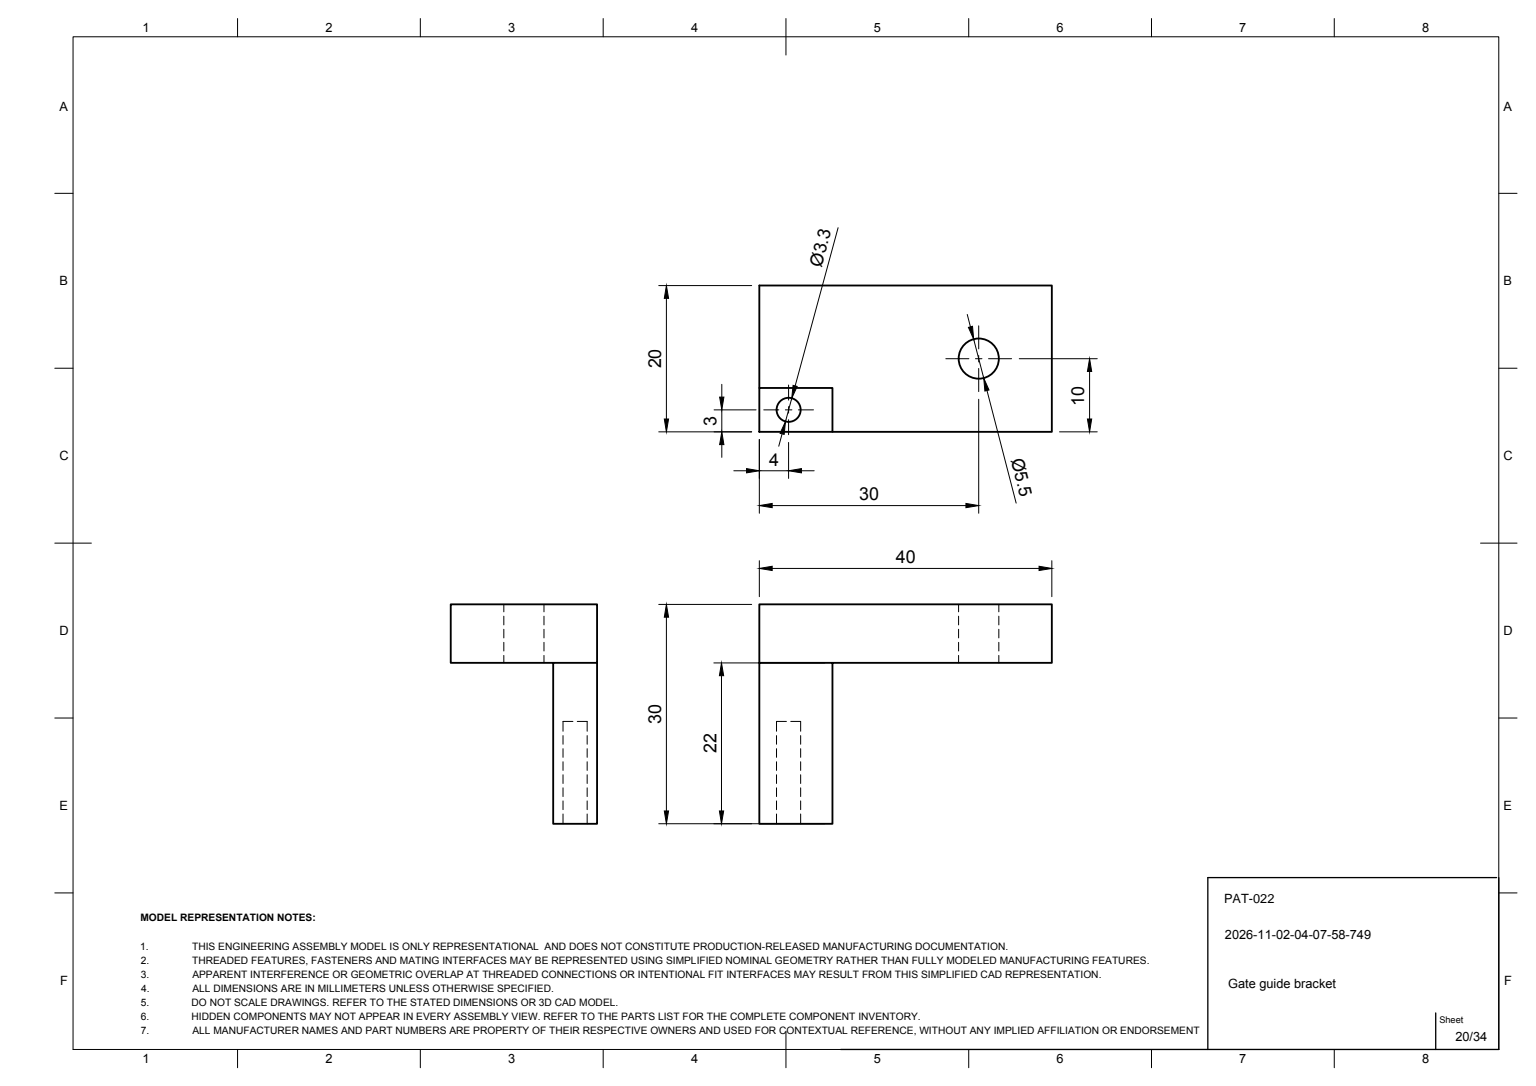
ISO-10303-21;
HEADER;
/* Generated by software containing ST-Developer
 * from STEP Tools, Inc. (www.steptools.com) 
 */

FILE_DESCRIPTION(
/* description */ ('Chute with adjustable gate'),
/* implementation_level */ '2;1');

FILE_NAME(
/* name */ 'Gate guide bracket.step',
/* time_stamp */ '2026-10-27T10:52:28-07:00',
/* author */ (''),
/* organization */ (''),
/* preprocessor_version */ 'ST-DEVELOPER v20.2',
/* originating_system */ 'Autodesk Translation Framework v15.17.0.0',
/* authorisation */ '');

FILE_SCHEMA (('AUTOMOTIVE_DESIGN { 1 0 10303 214 3 1 1 }'));
ENDSEC;

DATA;
#10=MECHANICAL_DESIGN_GEOMETRIC_PRESENTATION_REPRESENTATION('',(#429),#13094);
#365=SHAPE_REPRESENTATION_RELATIONSHIP('SRR','None',#13266,#397);
#397=ADVANCED_BREP_SHAPE_REPRESENTATION('',(#461),#13075);
#429=STYLED_ITEM('',(#13474),#461);
#461=MANIFOLD_SOLID_BREP('Body1',#7612);
#540=FACE_BOUND('',#1546,.T.);
#541=FACE_BOUND('',#1551,.T.);
#542=FACE_BOUND('',#1554,.T.);
#702=PLANE('',#8221);
#703=PLANE('',#8225);
#704=PLANE('',#8226);
#705=PLANE('',#8227);
#706=PLANE('',#8228);
#707=PLANE('',#8229);
#708=PLANE('',#8230);
#709=PLANE('',#8231);
#710=PLANE('',#8232);
#711=PLANE('',#8233);
#1060=FACE_OUTER_BOUND('',#1541,.T.);
#1061=FACE_OUTER_BOUND('',#1542,.T.);
#1062=FACE_OUTER_BOUND('',#1543,.T.);
#1063=FACE_OUTER_BOUND('',#1544,.T.);
#1064=FACE_OUTER_BOUND('',#1545,.T.);
#1065=FACE_OUTER_BOUND('',#1547,.T.);
#1066=FACE_OUTER_BOUND('',#1548,.T.);
#1067=FACE_OUTER_BOUND('',#1549,.T.);
#1068=FACE_OUTER_BOUND('',#1550,.T.);
#1069=FACE_OUTER_BOUND('',#1552,.T.);
#1070=FACE_OUTER_BOUND('',#1553,.T.);
#1071=FACE_OUTER_BOUND('',#1555,.T.);
#1541=EDGE_LOOP('',(#5834,#5835,#5836,#5837));
#1542=EDGE_LOOP('',(#5838));
#1543=EDGE_LOOP('',(#5839,#5840,#5841,#5842));
#1544=EDGE_LOOP('',(#5843,#5844,#5845,#5846));
#1545=EDGE_LOOP('',(#5847,#5848,#5849,#5850));
#1546=EDGE_LOOP('',(#5851));
#1547=EDGE_LOOP('',(#5852,#5853,#5854,#5855));
#1548=EDGE_LOOP('',(#5856,#5857,#5858,#5859,#5860,#5861));
#1549=EDGE_LOOP('',(#5862,#5863,#5864,#5865,#5866,#5867));
#1550=EDGE_LOOP('',(#5868,#5869,#5870,#5871));
#1551=EDGE_LOOP('',(#5872));
#1552=EDGE_LOOP('',(#5873,#5874,#5875,#5876));
#1553=EDGE_LOOP('',(#5877,#5878,#5879,#5880,#5881,#5882));
#1554=EDGE_LOOP('',(#5883));
#1555=EDGE_LOOP('',(#5884,#5885,#5886,#5887));
#2116=LINE('',#11607,#2893);
#2117=LINE('',#11614,#2894);
#2118=LINE('',#11619,#2895);
#2119=LINE('',#11621,#2896);
#2120=LINE('',#11623,#2897);
#2121=LINE('',#11624,#2898);
#2122=LINE('',#11627,#2899);
#2123=LINE('',#11629,#2900);
#2124=LINE('',#11630,#2901);
#2125=LINE('',#11633,#2902);
#2126=LINE('',#11634,#2903);
#2127=LINE('',#11637,#2904);
#2128=LINE('',#11639,#2905);
#2129=LINE('',#11641,#2906);
#2130=LINE('',#11642,#2907);
#2131=LINE('',#11645,#2908);
#2132=LINE('',#11647,#2909);
#2133=LINE('',#11648,#2910);
#2134=LINE('',#11651,#2911);
#2135=LINE('',#11652,#2912);
#2136=LINE('',#11655,#2913);
#2137=LINE('',#11656,#2914);
#2138=LINE('',#11658,#2915);
#2893=VECTOR('',#9422,0.164999999999999);
#2894=VECTOR('',#9431,0.274999999999999);
#2895=VECTOR('',#9436,1.);
#2896=VECTOR('',#9437,1.);
#2897=VECTOR('',#9438,1.);
#2898=VECTOR('',#9439,1.);
#2899=VECTOR('',#9442,1.);
#2900=VECTOR('',#9443,1.);
#2901=VECTOR('',#9444,1.);
#2902=VECTOR('',#9447,1.);
#2903=VECTOR('',#9448,1.);
#2904=VECTOR('',#9451,1.);
#2905=VECTOR('',#9452,1.);
#2906=VECTOR('',#9453,1.);
#2907=VECTOR('',#9454,1.);
#2908=VECTOR('',#9457,1.);
#2909=VECTOR('',#9458,1.);
#2910=VECTOR('',#9459,1.);
#2911=VECTOR('',#9462,1.);
#2912=VECTOR('',#9463,1.);
#2913=VECTOR('',#9466,1.);
#2914=VECTOR('',#9467,1.);
#2915=VECTOR('',#9470,1.);
#3482=CIRCLE('',#8219,0.164999999999999);
#3483=CIRCLE('',#8220,0.164999999999999);
#3484=CIRCLE('',#8223,0.274999999999999);
#3485=CIRCLE('',#8224,0.274999999999999);
#3809=VERTEX_POINT('',#11604);
#3810=VERTEX_POINT('',#11606);
#3811=VERTEX_POINT('',#11611);
#3812=VERTEX_POINT('',#11613);
#3813=VERTEX_POINT('',#11617);
#3814=VERTEX_POINT('',#11618);
#3815=VERTEX_POINT('',#11620);
#3816=VERTEX_POINT('',#11622);
#3817=VERTEX_POINT('',#11626);
#3818=VERTEX_POINT('',#11628);
#3819=VERTEX_POINT('',#11632);
#3820=VERTEX_POINT('',#11636);
#3821=VERTEX_POINT('',#11638);
#3822=VERTEX_POINT('',#11640);
#3823=VERTEX_POINT('',#11644);
#3824=VERTEX_POINT('',#11646);
#3825=VERTEX_POINT('',#11650);
#3826=VERTEX_POINT('',#11654);
#4550=EDGE_CURVE('',#3809,#3809,#3482,.T.);
#4551=EDGE_CURVE('',#3809,#3810,#2116,.T.);
#4552=EDGE_CURVE('',#3810,#3810,#3483,.T.);
#4553=EDGE_CURVE('',#3811,#3811,#3484,.T.);
#4554=EDGE_CURVE('',#3811,#3812,#2117,.T.);
#4555=EDGE_CURVE('',#3812,#3812,#3485,.T.);
#4556=EDGE_CURVE('',#3813,#3814,#2118,.T.);
#4557=EDGE_CURVE('',#3815,#3813,#2119,.T.);
#4558=EDGE_CURVE('',#3816,#3815,#2120,.T.);
#4559=EDGE_CURVE('',#3814,#3816,#2121,.T.);
#4560=EDGE_CURVE('',#3816,#3817,#2122,.T.);
#4561=EDGE_CURVE('',#3818,#3815,#2123,.T.);
#4562=EDGE_CURVE('',#3817,#3818,#2124,.T.);
#4563=EDGE_CURVE('',#3814,#3819,#2125,.T.);
#4564=EDGE_CURVE('',#3817,#3819,#2126,.T.);
#4565=EDGE_CURVE('',#3813,#3820,#2127,.T.);
#4566=EDGE_CURVE('',#3821,#3820,#2128,.T.);
#4567=EDGE_CURVE('',#3822,#3821,#2129,.T.);
#4568=EDGE_CURVE('',#3822,#3818,#2130,.T.);
#4569=EDGE_CURVE('',#3823,#3822,#2131,.T.);
#4570=EDGE_CURVE('',#3824,#3823,#2132,.T.);
#4571=EDGE_CURVE('',#3819,#3824,#2133,.T.);
#4572=EDGE_CURVE('',#3825,#3821,#2134,.T.);
#4573=EDGE_CURVE('',#3823,#3825,#2135,.T.);
#4574=EDGE_CURVE('',#3826,#3825,#2136,.T.);
#4575=EDGE_CURVE('',#3824,#3826,#2137,.T.);
#4576=EDGE_CURVE('',#3820,#3826,#2138,.T.);
#5834=ORIENTED_EDGE('',*,*,#4550,.F.);
#5835=ORIENTED_EDGE('',*,*,#4551,.T.);
#5836=ORIENTED_EDGE('',*,*,#4552,.T.);
#5837=ORIENTED_EDGE('',*,*,#4551,.F.);
#5838=ORIENTED_EDGE('',*,*,#4552,.F.);
#5839=ORIENTED_EDGE('',*,*,#4553,.F.);
#5840=ORIENTED_EDGE('',*,*,#4554,.T.);
#5841=ORIENTED_EDGE('',*,*,#4555,.F.);
#5842=ORIENTED_EDGE('',*,*,#4554,.F.);
#5843=ORIENTED_EDGE('',*,*,#4556,.F.);
#5844=ORIENTED_EDGE('',*,*,#4557,.F.);
#5845=ORIENTED_EDGE('',*,*,#4558,.F.);
#5846=ORIENTED_EDGE('',*,*,#4559,.F.);
#5847=ORIENTED_EDGE('',*,*,#4560,.F.);
#5848=ORIENTED_EDGE('',*,*,#4558,.T.);
#5849=ORIENTED_EDGE('',*,*,#4561,.F.);
#5850=ORIENTED_EDGE('',*,*,#4562,.F.);
#5851=ORIENTED_EDGE('',*,*,#4550,.T.);
#5852=ORIENTED_EDGE('',*,*,#4563,.F.);
#5853=ORIENTED_EDGE('',*,*,#4559,.T.);
#5854=ORIENTED_EDGE('',*,*,#4560,.T.);
#5855=ORIENTED_EDGE('',*,*,#4564,.T.);
#5856=ORIENTED_EDGE('',*,*,#4565,.T.);
#5857=ORIENTED_EDGE('',*,*,#4566,.F.);
#5858=ORIENTED_EDGE('',*,*,#4567,.F.);
#5859=ORIENTED_EDGE('',*,*,#4568,.T.);
#5860=ORIENTED_EDGE('',*,*,#4561,.T.);
#5861=ORIENTED_EDGE('',*,*,#4557,.T.);
#5862=ORIENTED_EDGE('',*,*,#4569,.F.);
#5863=ORIENTED_EDGE('',*,*,#4570,.F.);
#5864=ORIENTED_EDGE('',*,*,#4571,.F.);
#5865=ORIENTED_EDGE('',*,*,#4564,.F.);
#5866=ORIENTED_EDGE('',*,*,#4562,.T.);
#5867=ORIENTED_EDGE('',*,*,#4568,.F.);
#5868=ORIENTED_EDGE('',*,*,#4567,.T.);
#5869=ORIENTED_EDGE('',*,*,#4572,.F.);
#5870=ORIENTED_EDGE('',*,*,#4573,.F.);
#5871=ORIENTED_EDGE('',*,*,#4569,.T.);
#5872=ORIENTED_EDGE('',*,*,#4555,.T.);
#5873=ORIENTED_EDGE('',*,*,#4570,.T.);
#5874=ORIENTED_EDGE('',*,*,#4573,.T.);
#5875=ORIENTED_EDGE('',*,*,#4574,.F.);
#5876=ORIENTED_EDGE('',*,*,#4575,.F.);
#5877=ORIENTED_EDGE('',*,*,#4563,.T.);
#5878=ORIENTED_EDGE('',*,*,#4571,.T.);
#5879=ORIENTED_EDGE('',*,*,#4575,.T.);
#5880=ORIENTED_EDGE('',*,*,#4576,.F.);
#5881=ORIENTED_EDGE('',*,*,#4565,.F.);
#5882=ORIENTED_EDGE('',*,*,#4556,.T.);
#5883=ORIENTED_EDGE('',*,*,#4553,.T.);
#5884=ORIENTED_EDGE('',*,*,#4576,.T.);
#5885=ORIENTED_EDGE('',*,*,#4574,.T.);
#5886=ORIENTED_EDGE('',*,*,#4572,.T.);
#5887=ORIENTED_EDGE('',*,*,#4566,.T.);
#7140=CYLINDRICAL_SURFACE('',#8218,0.164999999999999);
#7141=CYLINDRICAL_SURFACE('',#8222,0.274999999999999);
#7328=ADVANCED_FACE('',(#1060),#7140,.F.);
#7329=ADVANCED_FACE('',(#1061),#702,.F.);
#7330=ADVANCED_FACE('',(#1062),#7141,.F.);
#7331=ADVANCED_FACE('',(#1063),#703,.T.);
#7332=ADVANCED_FACE('',(#1064,#540),#704,.T.);
#7333=ADVANCED_FACE('',(#1065),#705,.F.);
#7334=ADVANCED_FACE('',(#1066),#706,.T.);
#7335=ADVANCED_FACE('',(#1067),#707,.F.);
#7336=ADVANCED_FACE('',(#1068,#541),#708,.T.);
#7337=ADVANCED_FACE('',(#1069),#709,.T.);
#7338=ADVANCED_FACE('',(#1070,#542),#710,.T.);
#7339=ADVANCED_FACE('',(#1071),#711,.T.);
#7612=CLOSED_SHELL('',(#7328,#7329,#7330,#7331,#7332,#7333,#7334,#7335,
#7336,#7337,#7338,#7339));
#8217=AXIS2_PLACEMENT_3D('',#11602,#9416,#9417);
#8218=AXIS2_PLACEMENT_3D('',#11603,#9418,#9419);
#8219=AXIS2_PLACEMENT_3D('',#11605,#9420,#9421);
#8220=AXIS2_PLACEMENT_3D('',#11608,#9423,#9424);
#8221=AXIS2_PLACEMENT_3D('',#11609,#9425,#9426);
#8222=AXIS2_PLACEMENT_3D('',#11610,#9427,#9428);
#8223=AXIS2_PLACEMENT_3D('',#11612,#9429,#9430);
#8224=AXIS2_PLACEMENT_3D('',#11615,#9432,#9433);
#8225=AXIS2_PLACEMENT_3D('',#11616,#9434,#9435);
#8226=AXIS2_PLACEMENT_3D('',#11625,#9440,#9441);
#8227=AXIS2_PLACEMENT_3D('',#11631,#9445,#9446);
#8228=AXIS2_PLACEMENT_3D('',#11635,#9449,#9450);
#8229=AXIS2_PLACEMENT_3D('',#11643,#9455,#9456);
#8230=AXIS2_PLACEMENT_3D('',#11649,#9460,#9461);
#8231=AXIS2_PLACEMENT_3D('',#11653,#9464,#9465);
#8232=AXIS2_PLACEMENT_3D('',#11657,#9468,#9469);
#8233=AXIS2_PLACEMENT_3D('',#11659,#9471,#9472);
#9416=DIRECTION('axis',(0.,0.,1.));
#9417=DIRECTION('refdir',(1.,0.,0.));
#9418=DIRECTION('center_axis',(1.,0.,0.));
#9419=DIRECTION('ref_axis',(0.,0.,-1.));
#9420=DIRECTION('center_axis',(1.,0.,0.));
#9421=DIRECTION('ref_axis',(0.,0.,-1.));
#9422=DIRECTION('',(1.,0.,0.));
#9423=DIRECTION('center_axis',(1.,0.,0.));
#9424=DIRECTION('ref_axis',(0.,0.,-1.));
#9425=DIRECTION('center_axis',(1.,0.,0.));
#9426=DIRECTION('ref_axis',(0.,0.,-1.));
#9427=DIRECTION('center_axis',(1.,0.,0.));
#9428=DIRECTION('ref_axis',(0.,0.,-1.));
#9429=DIRECTION('center_axis',(1.,0.,0.));
#9430=DIRECTION('ref_axis',(0.,0.,-1.));
#9431=DIRECTION('',(1.,0.,0.));
#9432=DIRECTION('center_axis',(-1.,0.,0.));
#9433=DIRECTION('ref_axis',(0.,0.,-1.));
#9434=DIRECTION('center_axis',(0.,0.,1.));
#9435=DIRECTION('ref_axis',(1.,0.,0.));
#9436=DIRECTION('',(0.,-1.,0.));
#9437=DIRECTION('',(1.,0.,0.));
#9438=DIRECTION('',(0.,1.,0.));
#9439=DIRECTION('',(-1.,0.,0.));
#9440=DIRECTION('center_axis',(-1.,0.,0.));
#9441=DIRECTION('ref_axis',(0.,0.,1.));
#9442=DIRECTION('',(0.,0.,-1.));
#9443=DIRECTION('',(0.,0.,1.));
#9444=DIRECTION('',(0.,1.,0.));
#9445=DIRECTION('center_axis',(0.,1.,0.));
#9446=DIRECTION('ref_axis',(1.,0.,0.));
#9447=DIRECTION('',(0.,0.,-1.));
#9448=DIRECTION('',(1.,0.,0.));
#9449=DIRECTION('center_axis',(0.,1.,0.));
#9450=DIRECTION('ref_axis',(-1.,0.,0.));
#9451=DIRECTION('',(0.,0.,1.));
#9452=DIRECTION('',(-1.,0.,0.));
#9453=DIRECTION('',(0.,0.,1.));
#9454=DIRECTION('',(-1.,0.,0.));
#9455=DIRECTION('center_axis',(0.,0.,1.));
#9456=DIRECTION('ref_axis',(1.,0.,0.));
#9457=DIRECTION('',(0.,1.,0.));
#9458=DIRECTION('',(1.,0.,0.));
#9459=DIRECTION('',(0.,-1.,0.));
#9460=DIRECTION('center_axis',(1.,0.,0.));
#9461=DIRECTION('ref_axis',(0.,1.,0.));
#9462=DIRECTION('',(0.,1.,0.));
#9463=DIRECTION('',(0.,0.,1.));
#9464=DIRECTION('center_axis',(0.,-1.,0.));
#9465=DIRECTION('ref_axis',(1.,0.,0.));
#9466=DIRECTION('',(1.,0.,0.));
#9467=DIRECTION('',(0.,0.,1.));
#9468=DIRECTION('center_axis',(-1.,0.,0.));
#9469=DIRECTION('ref_axis',(0.,-1.,0.));
#9470=DIRECTION('',(0.,-1.,0.));
#9471=DIRECTION('center_axis',(0.,0.,1.));
#9472=DIRECTION('ref_axis',(1.,0.,0.));
#11602=CARTESIAN_POINT('',(0.,0.,0.));
#11603=CARTESIAN_POINT('Origin',(-1.1,-8.4,18.3));
#11604=CARTESIAN_POINT('',(-1.,-8.4,18.465));
#11605=CARTESIAN_POINT('Origin',(-1.,-8.4,18.3));
#11606=CARTESIAN_POINT('',(0.4,-8.4,18.465));
#11607=CARTESIAN_POINT('',(-1.1,-8.4,18.465));
#11608=CARTESIAN_POINT('Origin',(0.4,-8.4,18.3));
#11609=CARTESIAN_POINT('Origin',(0.4,-8.4,18.3));
#11610=CARTESIAN_POINT('Origin',(1.1,-11.,19.));
#11611=CARTESIAN_POINT('',(1.2,-11.,19.275));
#11612=CARTESIAN_POINT('Origin',(1.2,-11.,19.));
#11613=CARTESIAN_POINT('',(2.,-11.,19.275));
#11614=CARTESIAN_POINT('',(1.1,-11.,19.275));
#11615=CARTESIAN_POINT('Origin',(2.,-11.,19.));
#11616=CARTESIAN_POINT('Origin',(-1.,-9.,18.6));
#11617=CARTESIAN_POINT('',(1.2,-8.,18.6));
#11618=CARTESIAN_POINT('',(1.2,-9.,18.6));
#11619=CARTESIAN_POINT('',(1.2,-8.5,18.6));
#11620=CARTESIAN_POINT('',(-1.,-8.,18.6));
#11621=CARTESIAN_POINT('',(2.,-8.,18.6));
#11622=CARTESIAN_POINT('',(-1.,-9.,18.6));
#11623=CARTESIAN_POINT('',(-1.,-9.,18.6));
#11624=CARTESIAN_POINT('',(2.,-9.,18.6));
#11625=CARTESIAN_POINT('Origin',(-1.,-9.,18.));
#11626=CARTESIAN_POINT('',(-1.,-9.,18.));
#11627=CARTESIAN_POINT('',(-1.,-9.,18.6));
#11628=CARTESIAN_POINT('',(-1.,-8.,18.));
#11629=CARTESIAN_POINT('',(-1.,-8.,18.6));
#11630=CARTESIAN_POINT('',(-1.,-9.,18.));
#11631=CARTESIAN_POINT('Origin',(0.5,-9.,18.3));
#11632=CARTESIAN_POINT('',(1.2,-9.,18.));
#11633=CARTESIAN_POINT('',(1.2,-9.,18.15));
#11634=CARTESIAN_POINT('',(-1.,-9.,18.));
#11635=CARTESIAN_POINT('Origin',(2.,-8.,18.));
#11636=CARTESIAN_POINT('',(1.2,-8.,20.));
#11637=CARTESIAN_POINT('',(1.2,-8.,18.));
#11638=CARTESIAN_POINT('',(2.,-8.,20.));
#11639=CARTESIAN_POINT('',(2.,-8.,20.));
#11640=CARTESIAN_POINT('',(2.,-8.,18.));
#11641=CARTESIAN_POINT('',(2.,-8.,18.));
#11642=CARTESIAN_POINT('',(2.,-8.,18.));
#11643=CARTESIAN_POINT('Origin',(1.6,-10.,18.));
#11644=CARTESIAN_POINT('',(2.,-12.,18.));
#11645=CARTESIAN_POINT('',(2.,-12.,18.));
#11646=CARTESIAN_POINT('',(1.2,-12.,18.));
#11647=CARTESIAN_POINT('',(1.2,-12.,18.));
#11648=CARTESIAN_POINT('',(1.2,-8.,18.));
#11649=CARTESIAN_POINT('Origin',(2.,-12.,18.));
#11650=CARTESIAN_POINT('',(2.,-12.,20.));
#11651=CARTESIAN_POINT('',(2.,-12.,20.));
#11652=CARTESIAN_POINT('',(2.,-12.,18.));
#11653=CARTESIAN_POINT('Origin',(1.2,-12.,18.));
#11654=CARTESIAN_POINT('',(1.2,-12.,20.));
#11655=CARTESIAN_POINT('',(1.2,-12.,20.));
#11656=CARTESIAN_POINT('',(1.2,-12.,18.));
#11657=CARTESIAN_POINT('Origin',(1.2,-8.,18.));
#11658=CARTESIAN_POINT('',(1.2,-8.,20.));
#11659=CARTESIAN_POINT('Origin',(1.6,-10.,20.));
#13038=UNCERTAINTY_MEASURE_WITH_UNIT(LENGTH_MEASURE(0.001),#13095,
'DISTANCE_ACCURACY_VALUE',
'Maximum model space distance between geometric entities at asserted c
onnectivities');
#13057=UNCERTAINTY_MEASURE_WITH_UNIT(LENGTH_MEASURE(0.001),#13095,
'DISTANCE_ACCURACY_VALUE',
'Maximum model space distance between geometric entities at asserted c
onnectivities');
#13075=(
GEOMETRIC_REPRESENTATION_CONTEXT(3)
GLOBAL_UNCERTAINTY_ASSIGNED_CONTEXT((#13038))
GLOBAL_UNIT_ASSIGNED_CONTEXT((#13095,#13097,#13098))
REPRESENTATION_CONTEXT('','3D')
);
#13094=(
GEOMETRIC_REPRESENTATION_CONTEXT(3)
GLOBAL_UNCERTAINTY_ASSIGNED_CONTEXT((#13057))
GLOBAL_UNIT_ASSIGNED_CONTEXT((#13095,#13097,#13098))
REPRESENTATION_CONTEXT('','3D')
);
#13095=(
LENGTH_UNIT()
NAMED_UNIT(*)
SI_UNIT(.CENTI.,.METRE.)
);
#13097=(
NAMED_UNIT(*)
PLANE_ANGLE_UNIT()
SI_UNIT($,.RADIAN.)
);
#13098=(
NAMED_UNIT(*)
SI_UNIT($,.STERADIAN.)
SOLID_ANGLE_UNIT()
);
#13116=SHAPE_DEFINITION_REPRESENTATION(#13152,#13266);
#13152=PRODUCT_DEFINITION_SHAPE('',$,#13303);
#13266=SHAPE_REPRESENTATION('',(#8217),#13075);
#13285=PRODUCT_DEFINITION_CONTEXT('part definition',#13395,'design');
#13303=PRODUCT_DEFINITION('Gate guide bracket','Gate guide bracket',#13339,
#13285);
#13339=PRODUCT_DEFINITION_FORMATION('',$,#13414);
#13395=APPLICATION_CONTEXT(
'Core Data for Automotive Mechanical Design Process');
#13396=PRODUCT_CONTEXT('part definition',#13395,'mechanical');
#13414=PRODUCT('Gate guide bracket','Gate guide bracket',
'Gate guide bracket',(#13396));
#13468=COLOUR_RGB('Dark Blue',0.08,0.2,0.34);
#13469=FILL_AREA_STYLE_COLOUR('',#13468);
#13470=FILL_AREA_STYLE('',(#13469));
#13471=SURFACE_STYLE_FILL_AREA(#13470);
#13472=SURFACE_SIDE_STYLE('',(#13471));
#13473=SURFACE_STYLE_USAGE(.BOTH.,#13472);
#13474=PRESENTATION_STYLE_ASSIGNMENT((#13473));
ENDSEC;
END-ISO-10303-21;
